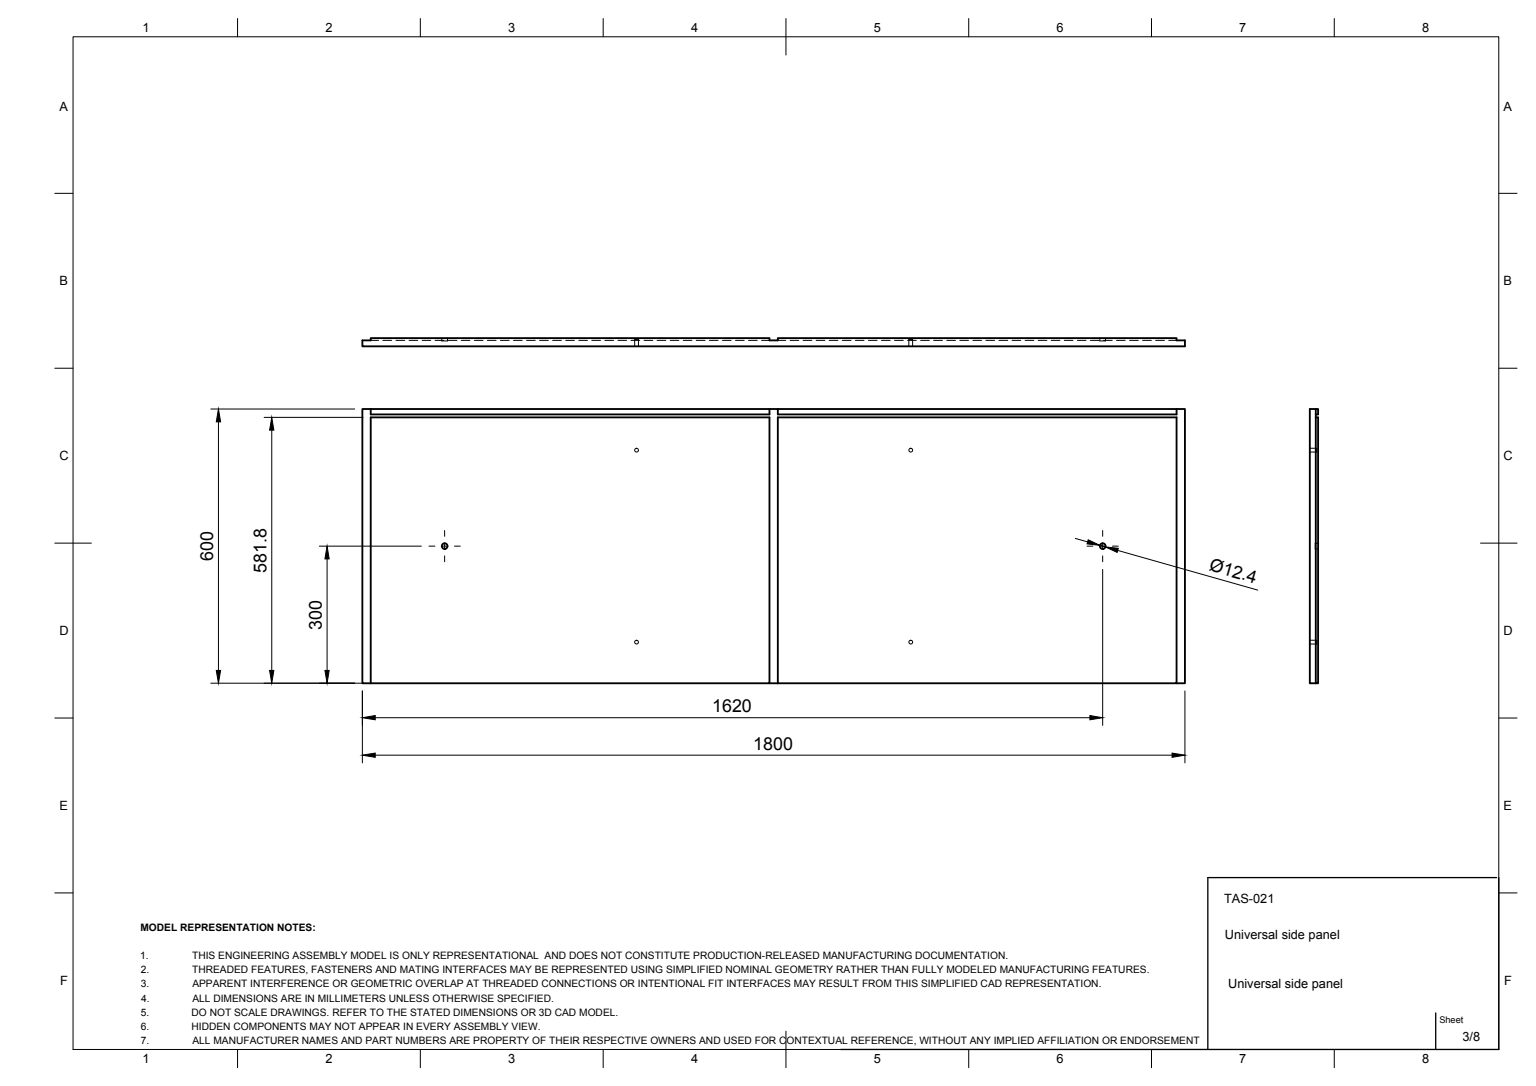
ISO-10303-21;
HEADER;
/* Generated by software containing ST-Developer
 * from STEP Tools, Inc. (www.steptools.com) 
 */

FILE_DESCRIPTION(
/* description */ (''),
/* implementation_level */ '2;1');

FILE_NAME(
/* name */ 'Universal side panel.step',
/* time_stamp */ '2026-11-15T17:48:08-08:00',
/* author */ (''),
/* organization */ (''),
/* preprocessor_version */ 'ST-DEVELOPER v20.2',
/* originating_system */ 'Autodesk Translation Framework v15.17.0.0',
/* authorisation */ '');

FILE_SCHEMA (('AUTOMOTIVE_DESIGN { 1 0 10303 214 3 1 1 }'));
ENDSEC;

DATA;
#10=MECHANICAL_DESIGN_GEOMETRIC_PRESENTATION_REPRESENTATION('',(#139),#2097);
#127=SHAPE_REPRESENTATION_RELATIONSHIP('SRR','None',#2146,#133);
#133=ADVANCED_BREP_SHAPE_REPRESENTATION('',(#145),#2091);
#139=STYLED_ITEM('',(#2185),#145);
#145=MANIFOLD_SOLID_BREP('Body1',#1193);
#151=FACE_BOUND('',#301,.T.);
#152=FACE_BOUND('',#308,.T.);
#153=FACE_BOUND('',#316,.T.);
#154=FACE_BOUND('',#317,.T.);
#155=FACE_BOUND('',#318,.T.);
#156=FACE_BOUND('',#319,.T.);
#159=PLANE('',#1271);
#160=PLANE('',#1275);
#161=PLANE('',#1279);
#162=PLANE('',#1283);
#163=PLANE('',#1287);
#164=PLANE('',#1291);
#165=PLANE('',#1292);
#166=PLANE('',#1293);
#167=PLANE('',#1294);
#168=PLANE('',#1295);
#169=PLANE('',#1296);
#170=PLANE('',#1297);
#171=PLANE('',#1298);
#172=PLANE('',#1299);
#173=PLANE('',#1300);
#174=PLANE('',#1301);
#175=PLANE('',#1302);
#176=PLANE('',#1303);
#177=PLANE('',#1304);
#178=PLANE('',#1305);
#179=PLANE('',#1306);
#180=PLANE('',#1307);
#181=PLANE('',#1308);
#182=PLANE('',#1309);
#183=PLANE('',#1310);
#184=PLANE('',#1311);
#185=PLANE('',#1312);
#186=PLANE('',#1313);
#215=FACE_OUTER_BOUND('',#281,.T.);
#216=FACE_OUTER_BOUND('',#282,.T.);
#217=FACE_OUTER_BOUND('',#283,.T.);
#218=FACE_OUTER_BOUND('',#284,.T.);
#219=FACE_OUTER_BOUND('',#285,.T.);
#220=FACE_OUTER_BOUND('',#286,.T.);
#221=FACE_OUTER_BOUND('',#287,.T.);
#222=FACE_OUTER_BOUND('',#288,.T.);
#223=FACE_OUTER_BOUND('',#289,.T.);
#224=FACE_OUTER_BOUND('',#290,.T.);
#225=FACE_OUTER_BOUND('',#291,.T.);
#226=FACE_OUTER_BOUND('',#292,.T.);
#227=FACE_OUTER_BOUND('',#293,.T.);
#228=FACE_OUTER_BOUND('',#294,.T.);
#229=FACE_OUTER_BOUND('',#295,.T.);
#230=FACE_OUTER_BOUND('',#296,.T.);
#231=FACE_OUTER_BOUND('',#297,.T.);
#232=FACE_OUTER_BOUND('',#298,.T.);
#233=FACE_OUTER_BOUND('',#299,.T.);
#234=FACE_OUTER_BOUND('',#300,.T.);
#235=FACE_OUTER_BOUND('',#302,.T.);
#236=FACE_OUTER_BOUND('',#303,.T.);
#237=FACE_OUTER_BOUND('',#304,.T.);
#238=FACE_OUTER_BOUND('',#305,.T.);
#239=FACE_OUTER_BOUND('',#306,.T.);
#240=FACE_OUTER_BOUND('',#307,.T.);
#241=FACE_OUTER_BOUND('',#309,.T.);
#242=FACE_OUTER_BOUND('',#310,.T.);
#243=FACE_OUTER_BOUND('',#311,.T.);
#244=FACE_OUTER_BOUND('',#312,.T.);
#245=FACE_OUTER_BOUND('',#313,.T.);
#246=FACE_OUTER_BOUND('',#314,.T.);
#247=FACE_OUTER_BOUND('',#315,.T.);
#248=FACE_OUTER_BOUND('',#320,.T.);
#281=EDGE_LOOP('',(#841,#842,#843,#844));
#282=EDGE_LOOP('',(#845));
#283=EDGE_LOOP('',(#846,#847,#848,#849));
#284=EDGE_LOOP('',(#850));
#285=EDGE_LOOP('',(#851,#852,#853,#854));
#286=EDGE_LOOP('',(#855));
#287=EDGE_LOOP('',(#856,#857,#858,#859));
#288=EDGE_LOOP('',(#860));
#289=EDGE_LOOP('',(#861,#862,#863,#864));
#290=EDGE_LOOP('',(#865));
#291=EDGE_LOOP('',(#866,#867,#868,#869));
#292=EDGE_LOOP('',(#870));
#293=EDGE_LOOP('',(#871,#872,#873,#874));
#294=EDGE_LOOP('',(#875,#876,#877,#878));
#295=EDGE_LOOP('',(#879,#880,#881,#882));
#296=EDGE_LOOP('',(#883,#884,#885,#886));
#297=EDGE_LOOP('',(#887,#888,#889,#890,#891,#892,#893,#894,#895,#896,#897,
#898,#899,#900,#901,#902,#903,#904,#905,#906));
#298=EDGE_LOOP('',(#907,#908,#909,#910));
#299=EDGE_LOOP('',(#911,#912,#913,#914));
#300=EDGE_LOOP('',(#915,#916,#917,#918));
#301=EDGE_LOOP('',(#919));
#302=EDGE_LOOP('',(#920,#921,#922,#923));
#303=EDGE_LOOP('',(#924,#925,#926,#927));
#304=EDGE_LOOP('',(#928,#929,#930,#931));
#305=EDGE_LOOP('',(#932,#933,#934,#935));
#306=EDGE_LOOP('',(#936,#937,#938,#939));
#307=EDGE_LOOP('',(#940,#941,#942,#943));
#308=EDGE_LOOP('',(#944));
#309=EDGE_LOOP('',(#945,#946,#947,#948));
#310=EDGE_LOOP('',(#949,#950,#951,#952));
#311=EDGE_LOOP('',(#953,#954,#955,#956));
#312=EDGE_LOOP('',(#957,#958,#959,#960,#961,#962,#963,#964,#965,#966,#967,
#968));
#313=EDGE_LOOP('',(#969,#970,#971,#972));
#314=EDGE_LOOP('',(#973,#974,#975,#976,#977,#978,#979,#980,#981,#982,#983,
#984));
#315=EDGE_LOOP('',(#985,#986,#987,#988));
#316=EDGE_LOOP('',(#989));
#317=EDGE_LOOP('',(#990));
#318=EDGE_LOOP('',(#991));
#319=EDGE_LOOP('',(#992));
#320=EDGE_LOOP('',(#993,#994,#995,#996));
#355=LINE('',#1756,#473);
#356=LINE('',#1763,#474);
#357=LINE('',#1770,#475);
#358=LINE('',#1777,#476);
#359=LINE('',#1784,#477);
#360=LINE('',#1791,#478);
#361=LINE('',#1797,#479);
#362=LINE('',#1799,#480);
#363=LINE('',#1801,#481);
#364=LINE('',#1802,#482);
#365=LINE('',#1806,#483);
#366=LINE('',#1808,#484);
#367=LINE('',#1810,#485);
#368=LINE('',#1811,#486);
#369=LINE('',#1815,#487);
#370=LINE('',#1817,#488);
#371=LINE('',#1819,#489);
#372=LINE('',#1820,#490);
#373=LINE('',#1824,#491);
#374=LINE('',#1826,#492);
#375=LINE('',#1828,#493);
#376=LINE('',#1829,#494);
#377=LINE('',#1832,#495);
#378=LINE('',#1834,#496);
#379=LINE('',#1836,#497);
#380=LINE('',#1838,#498);
#381=LINE('',#1839,#499);
#382=LINE('',#1841,#500);
#383=LINE('',#1843,#501);
#384=LINE('',#1844,#502);
#385=LINE('',#1846,#503);
#386=LINE('',#1848,#504);
#387=LINE('',#1850,#505);
#388=LINE('',#1852,#506);
#389=LINE('',#1853,#507);
#390=LINE('',#1855,#508);
#391=LINE('',#1857,#509);
#392=LINE('',#1858,#510);
#393=LINE('',#1861,#511);
#394=LINE('',#1862,#512);
#395=LINE('',#1865,#513);
#396=LINE('',#1866,#514);
#397=LINE('',#1869,#515);
#398=LINE('',#1870,#516);
#399=LINE('',#1873,#517);
#400=LINE('',#1874,#518);
#401=LINE('',#1876,#519);
#402=LINE('',#1878,#520);
#403=LINE('',#1881,#521);
#404=LINE('',#1882,#522);
#405=LINE('',#1885,#523);
#406=LINE('',#1886,#524);
#407=LINE('',#1889,#525);
#408=LINE('',#1890,#526);
#409=LINE('',#1893,#527);
#410=LINE('',#1894,#528);
#411=LINE('',#1896,#529);
#412=LINE('',#1898,#530);
#413=LINE('',#1901,#531);
#414=LINE('',#1903,#532);
#415=LINE('',#1904,#533);
#416=LINE('',#1907,#534);
#417=LINE('',#1908,#535);
#418=LINE('',#1911,#536);
#419=LINE('',#1912,#537);
#420=LINE('',#1914,#538);
#473=VECTOR('',#1396,0.409999999999997);
#474=VECTOR('',#1405,0.409999999999997);
#475=VECTOR('',#1414,0.409999999999997);
#476=VECTOR('',#1423,0.409999999999997);
#477=VECTOR('',#1432,0.620000000000001);
#478=VECTOR('',#1441,0.620000000000005);
#479=VECTOR('',#1448,1.);
#480=VECTOR('',#1449,1.);
#481=VECTOR('',#1450,1.);
#482=VECTOR('',#1451,1.);
#483=VECTOR('',#1454,1.);
#484=VECTOR('',#1455,1.);
#485=VECTOR('',#1456,1.);
#486=VECTOR('',#1457,1.);
#487=VECTOR('',#1460,1.);
#488=VECTOR('',#1461,1.);
#489=VECTOR('',#1462,1.);
#490=VECTOR('',#1463,1.);
#491=VECTOR('',#1466,1.);
#492=VECTOR('',#1467,1.);
#493=VECTOR('',#1468,1.);
#494=VECTOR('',#1469,1.);
#495=VECTOR('',#1472,1.);
#496=VECTOR('',#1473,1.);
#497=VECTOR('',#1474,1.);
#498=VECTOR('',#1475,1.);
#499=VECTOR('',#1476,1.);
#500=VECTOR('',#1477,1.);
#501=VECTOR('',#1478,1.);
#502=VECTOR('',#1479,1.);
#503=VECTOR('',#1480,1.);
#504=VECTOR('',#1481,1.);
#505=VECTOR('',#1482,1.);
#506=VECTOR('',#1483,1.);
#507=VECTOR('',#1484,1.);
#508=VECTOR('',#1485,1.);
#509=VECTOR('',#1486,1.);
#510=VECTOR('',#1487,1.);
#511=VECTOR('',#1490,1.);
#512=VECTOR('',#1491,1.);
#513=VECTOR('',#1494,1.);
#514=VECTOR('',#1495,1.);
#515=VECTOR('',#1498,1.);
#516=VECTOR('',#1499,1.);
#517=VECTOR('',#1502,1.);
#518=VECTOR('',#1503,1.);
#519=VECTOR('',#1506,1.);
#520=VECTOR('',#1509,1.);
#521=VECTOR('',#1512,1.);
#522=VECTOR('',#1513,1.);
#523=VECTOR('',#1516,1.);
#524=VECTOR('',#1517,1.);
#525=VECTOR('',#1520,1.);
#526=VECTOR('',#1521,1.);
#527=VECTOR('',#1524,1.);
#528=VECTOR('',#1525,1.);
#529=VECTOR('',#1528,1.);
#530=VECTOR('',#1531,1.);
#531=VECTOR('',#1534,1.);
#532=VECTOR('',#1535,1.);
#533=VECTOR('',#1536,1.);
#534=VECTOR('',#1539,1.);
#535=VECTOR('',#1540,1.);
#536=VECTOR('',#1543,1.);
#537=VECTOR('',#1544,1.);
#538=VECTOR('',#1547,1.);
#591=CIRCLE('',#1269,0.409999999999997);
#592=CIRCLE('',#1270,0.409999999999997);
#593=CIRCLE('',#1273,0.409999999999997);
#594=CIRCLE('',#1274,0.409999999999997);
#595=CIRCLE('',#1277,0.409999999999997);
#596=CIRCLE('',#1278,0.409999999999997);
#597=CIRCLE('',#1281,0.409999999999997);
#598=CIRCLE('',#1282,0.409999999999997);
#599=CIRCLE('',#1285,0.620000000000001);
#600=CIRCLE('',#1286,0.620000000000001);
#601=CIRCLE('',#1289,0.620000000000005);
#602=CIRCLE('',#1290,0.620000000000005);
#611=VERTEX_POINT('',#1753);
#612=VERTEX_POINT('',#1755);
#613=VERTEX_POINT('',#1760);
#614=VERTEX_POINT('',#1762);
#615=VERTEX_POINT('',#1767);
#616=VERTEX_POINT('',#1769);
#617=VERTEX_POINT('',#1774);
#618=VERTEX_POINT('',#1776);
#619=VERTEX_POINT('',#1781);
#620=VERTEX_POINT('',#1783);
#621=VERTEX_POINT('',#1788);
#622=VERTEX_POINT('',#1790);
#623=VERTEX_POINT('',#1795);
#624=VERTEX_POINT('',#1796);
#625=VERTEX_POINT('',#1798);
#626=VERTEX_POINT('',#1800);
#627=VERTEX_POINT('',#1804);
#628=VERTEX_POINT('',#1805);
#629=VERTEX_POINT('',#1807);
#630=VERTEX_POINT('',#1809);
#631=VERTEX_POINT('',#1813);
#632=VERTEX_POINT('',#1814);
#633=VERTEX_POINT('',#1816);
#634=VERTEX_POINT('',#1818);
#635=VERTEX_POINT('',#1822);
#636=VERTEX_POINT('',#1823);
#637=VERTEX_POINT('',#1825);
#638=VERTEX_POINT('',#1827);
#639=VERTEX_POINT('',#1831);
#640=VERTEX_POINT('',#1833);
#641=VERTEX_POINT('',#1835);
#642=VERTEX_POINT('',#1837);
#643=VERTEX_POINT('',#1840);
#644=VERTEX_POINT('',#1842);
#645=VERTEX_POINT('',#1845);
#646=VERTEX_POINT('',#1847);
#647=VERTEX_POINT('',#1849);
#648=VERTEX_POINT('',#1851);
#649=VERTEX_POINT('',#1854);
#650=VERTEX_POINT('',#1856);
#651=VERTEX_POINT('',#1860);
#652=VERTEX_POINT('',#1864);
#653=VERTEX_POINT('',#1868);
#654=VERTEX_POINT('',#1872);
#655=VERTEX_POINT('',#1880);
#656=VERTEX_POINT('',#1884);
#657=VERTEX_POINT('',#1888);
#658=VERTEX_POINT('',#1892);
#659=VERTEX_POINT('',#1900);
#660=VERTEX_POINT('',#1902);
#661=VERTEX_POINT('',#1906);
#662=VERTEX_POINT('',#1910);
#703=EDGE_CURVE('',#611,#611,#591,.T.);
#704=EDGE_CURVE('',#611,#612,#355,.T.);
#705=EDGE_CURVE('',#612,#612,#592,.T.);
#706=EDGE_CURVE('',#613,#613,#593,.T.);
#707=EDGE_CURVE('',#613,#614,#356,.T.);
#708=EDGE_CURVE('',#614,#614,#594,.T.);
#709=EDGE_CURVE('',#615,#615,#595,.T.);
#710=EDGE_CURVE('',#615,#616,#357,.T.);
#711=EDGE_CURVE('',#616,#616,#596,.T.);
#712=EDGE_CURVE('',#617,#617,#597,.T.);
#713=EDGE_CURVE('',#617,#618,#358,.T.);
#714=EDGE_CURVE('',#618,#618,#598,.T.);
#715=EDGE_CURVE('',#619,#619,#599,.T.);
#716=EDGE_CURVE('',#619,#620,#359,.T.);
#717=EDGE_CURVE('',#620,#620,#600,.T.);
#718=EDGE_CURVE('',#621,#621,#601,.T.);
#719=EDGE_CURVE('',#621,#622,#360,.T.);
#720=EDGE_CURVE('',#622,#622,#602,.T.);
#721=EDGE_CURVE('',#623,#624,#361,.T.);
#722=EDGE_CURVE('',#625,#623,#362,.T.);
#723=EDGE_CURVE('',#626,#625,#363,.T.);
#724=EDGE_CURVE('',#624,#626,#364,.T.);
#725=EDGE_CURVE('',#627,#628,#365,.T.);
#726=EDGE_CURVE('',#629,#627,#366,.T.);
#727=EDGE_CURVE('',#630,#629,#367,.T.);
#728=EDGE_CURVE('',#628,#630,#368,.T.);
#729=EDGE_CURVE('',#631,#632,#369,.T.);
#730=EDGE_CURVE('',#633,#631,#370,.T.);
#731=EDGE_CURVE('',#634,#633,#371,.T.);
#732=EDGE_CURVE('',#634,#632,#372,.T.);
#733=EDGE_CURVE('',#635,#636,#373,.T.);
#734=EDGE_CURVE('',#637,#635,#374,.T.);
#735=EDGE_CURVE('',#638,#637,#375,.T.);
#736=EDGE_CURVE('',#638,#636,#376,.T.);
#737=EDGE_CURVE('',#639,#627,#377,.T.);
#738=EDGE_CURVE('',#640,#639,#378,.T.);
#739=EDGE_CURVE('',#641,#640,#379,.T.);
#740=EDGE_CURVE('',#642,#641,#380,.T.);
#741=EDGE_CURVE('',#636,#642,#381,.T.);
#742=EDGE_CURVE('',#638,#643,#382,.T.);
#743=EDGE_CURVE('',#644,#643,#383,.T.);
#744=EDGE_CURVE('',#632,#644,#384,.T.);
#745=EDGE_CURVE('',#634,#645,#385,.T.);
#746=EDGE_CURVE('',#646,#645,#386,.T.);
#747=EDGE_CURVE('',#647,#646,#387,.T.);
#748=EDGE_CURVE('',#648,#647,#388,.T.);
#749=EDGE_CURVE('',#648,#625,#389,.T.);
#750=EDGE_CURVE('',#649,#623,#390,.T.);
#751=EDGE_CURVE('',#650,#649,#391,.T.);
#752=EDGE_CURVE('',#650,#629,#392,.T.);
#753=EDGE_CURVE('',#651,#642,#393,.T.);
#754=EDGE_CURVE('',#635,#651,#394,.T.);
#755=EDGE_CURVE('',#652,#628,#395,.T.);
#756=EDGE_CURVE('',#639,#652,#396,.T.);
#757=EDGE_CURVE('',#653,#651,#397,.T.);
#758=EDGE_CURVE('',#653,#637,#398,.T.);
#759=EDGE_CURVE('',#630,#654,#399,.T.);
#760=EDGE_CURVE('',#654,#652,#400,.T.);
#761=EDGE_CURVE('',#643,#653,#401,.T.);
#762=EDGE_CURVE('',#654,#650,#402,.T.);
#763=EDGE_CURVE('',#655,#644,#403,.T.);
#764=EDGE_CURVE('',#631,#655,#404,.T.);
#765=EDGE_CURVE('',#656,#624,#405,.T.);
#766=EDGE_CURVE('',#649,#656,#406,.T.);
#767=EDGE_CURVE('',#657,#655,#407,.T.);
#768=EDGE_CURVE('',#657,#633,#408,.T.);
#769=EDGE_CURVE('',#626,#658,#409,.T.);
#770=EDGE_CURVE('',#658,#656,#410,.T.);
#771=EDGE_CURVE('',#645,#657,#411,.T.);
#772=EDGE_CURVE('',#658,#648,#412,.T.);
#773=EDGE_CURVE('',#647,#659,#413,.T.);
#774=EDGE_CURVE('',#659,#660,#414,.T.);
#775=EDGE_CURVE('',#640,#660,#415,.T.);
#776=EDGE_CURVE('',#661,#646,#416,.T.);
#777=EDGE_CURVE('',#659,#661,#417,.T.);
#778=EDGE_CURVE('',#662,#641,#418,.T.);
#779=EDGE_CURVE('',#661,#662,#419,.T.);
#780=EDGE_CURVE('',#660,#662,#420,.T.);
#841=ORIENTED_EDGE('',*,*,#703,.F.);
#842=ORIENTED_EDGE('',*,*,#704,.T.);
#843=ORIENTED_EDGE('',*,*,#705,.T.);
#844=ORIENTED_EDGE('',*,*,#704,.F.);
#845=ORIENTED_EDGE('',*,*,#705,.F.);
#846=ORIENTED_EDGE('',*,*,#706,.F.);
#847=ORIENTED_EDGE('',*,*,#707,.T.);
#848=ORIENTED_EDGE('',*,*,#708,.T.);
#849=ORIENTED_EDGE('',*,*,#707,.F.);
#850=ORIENTED_EDGE('',*,*,#708,.F.);
#851=ORIENTED_EDGE('',*,*,#709,.F.);
#852=ORIENTED_EDGE('',*,*,#710,.T.);
#853=ORIENTED_EDGE('',*,*,#711,.T.);
#854=ORIENTED_EDGE('',*,*,#710,.F.);
#855=ORIENTED_EDGE('',*,*,#711,.F.);
#856=ORIENTED_EDGE('',*,*,#712,.F.);
#857=ORIENTED_EDGE('',*,*,#713,.T.);
#858=ORIENTED_EDGE('',*,*,#714,.T.);
#859=ORIENTED_EDGE('',*,*,#713,.F.);
#860=ORIENTED_EDGE('',*,*,#714,.F.);
#861=ORIENTED_EDGE('',*,*,#715,.F.);
#862=ORIENTED_EDGE('',*,*,#716,.T.);
#863=ORIENTED_EDGE('',*,*,#717,.T.);
#864=ORIENTED_EDGE('',*,*,#716,.F.);
#865=ORIENTED_EDGE('',*,*,#717,.F.);
#866=ORIENTED_EDGE('',*,*,#718,.F.);
#867=ORIENTED_EDGE('',*,*,#719,.T.);
#868=ORIENTED_EDGE('',*,*,#720,.T.);
#869=ORIENTED_EDGE('',*,*,#719,.F.);
#870=ORIENTED_EDGE('',*,*,#720,.F.);
#871=ORIENTED_EDGE('',*,*,#721,.F.);
#872=ORIENTED_EDGE('',*,*,#722,.F.);
#873=ORIENTED_EDGE('',*,*,#723,.F.);
#874=ORIENTED_EDGE('',*,*,#724,.F.);
#875=ORIENTED_EDGE('',*,*,#725,.F.);
#876=ORIENTED_EDGE('',*,*,#726,.F.);
#877=ORIENTED_EDGE('',*,*,#727,.F.);
#878=ORIENTED_EDGE('',*,*,#728,.F.);
#879=ORIENTED_EDGE('',*,*,#729,.F.);
#880=ORIENTED_EDGE('',*,*,#730,.F.);
#881=ORIENTED_EDGE('',*,*,#731,.F.);
#882=ORIENTED_EDGE('',*,*,#732,.T.);
#883=ORIENTED_EDGE('',*,*,#733,.F.);
#884=ORIENTED_EDGE('',*,*,#734,.F.);
#885=ORIENTED_EDGE('',*,*,#735,.F.);
#886=ORIENTED_EDGE('',*,*,#736,.T.);
#887=ORIENTED_EDGE('',*,*,#737,.F.);
#888=ORIENTED_EDGE('',*,*,#738,.F.);
#889=ORIENTED_EDGE('',*,*,#739,.F.);
#890=ORIENTED_EDGE('',*,*,#740,.F.);
#891=ORIENTED_EDGE('',*,*,#741,.F.);
#892=ORIENTED_EDGE('',*,*,#736,.F.);
#893=ORIENTED_EDGE('',*,*,#742,.T.);
#894=ORIENTED_EDGE('',*,*,#743,.F.);
#895=ORIENTED_EDGE('',*,*,#744,.F.);
#896=ORIENTED_EDGE('',*,*,#732,.F.);
#897=ORIENTED_EDGE('',*,*,#745,.T.);
#898=ORIENTED_EDGE('',*,*,#746,.F.);
#899=ORIENTED_EDGE('',*,*,#747,.F.);
#900=ORIENTED_EDGE('',*,*,#748,.F.);
#901=ORIENTED_EDGE('',*,*,#749,.T.);
#902=ORIENTED_EDGE('',*,*,#722,.T.);
#903=ORIENTED_EDGE('',*,*,#750,.F.);
#904=ORIENTED_EDGE('',*,*,#751,.F.);
#905=ORIENTED_EDGE('',*,*,#752,.T.);
#906=ORIENTED_EDGE('',*,*,#726,.T.);
#907=ORIENTED_EDGE('',*,*,#733,.T.);
#908=ORIENTED_EDGE('',*,*,#741,.T.);
#909=ORIENTED_EDGE('',*,*,#753,.F.);
#910=ORIENTED_EDGE('',*,*,#754,.F.);
#911=ORIENTED_EDGE('',*,*,#725,.T.);
#912=ORIENTED_EDGE('',*,*,#755,.F.);
#913=ORIENTED_EDGE('',*,*,#756,.F.);
#914=ORIENTED_EDGE('',*,*,#737,.T.);
#915=ORIENTED_EDGE('',*,*,#734,.T.);
#916=ORIENTED_EDGE('',*,*,#754,.T.);
#917=ORIENTED_EDGE('',*,*,#757,.F.);
#918=ORIENTED_EDGE('',*,*,#758,.T.);
#919=ORIENTED_EDGE('',*,*,#718,.T.);
#920=ORIENTED_EDGE('',*,*,#728,.T.);
#921=ORIENTED_EDGE('',*,*,#759,.T.);
#922=ORIENTED_EDGE('',*,*,#760,.T.);
#923=ORIENTED_EDGE('',*,*,#755,.T.);
#924=ORIENTED_EDGE('',*,*,#735,.T.);
#925=ORIENTED_EDGE('',*,*,#758,.F.);
#926=ORIENTED_EDGE('',*,*,#761,.F.);
#927=ORIENTED_EDGE('',*,*,#742,.F.);
#928=ORIENTED_EDGE('',*,*,#727,.T.);
#929=ORIENTED_EDGE('',*,*,#752,.F.);
#930=ORIENTED_EDGE('',*,*,#762,.F.);
#931=ORIENTED_EDGE('',*,*,#759,.F.);
#932=ORIENTED_EDGE('',*,*,#729,.T.);
#933=ORIENTED_EDGE('',*,*,#744,.T.);
#934=ORIENTED_EDGE('',*,*,#763,.F.);
#935=ORIENTED_EDGE('',*,*,#764,.F.);
#936=ORIENTED_EDGE('',*,*,#721,.T.);
#937=ORIENTED_EDGE('',*,*,#765,.F.);
#938=ORIENTED_EDGE('',*,*,#766,.F.);
#939=ORIENTED_EDGE('',*,*,#750,.T.);
#940=ORIENTED_EDGE('',*,*,#730,.T.);
#941=ORIENTED_EDGE('',*,*,#764,.T.);
#942=ORIENTED_EDGE('',*,*,#767,.F.);
#943=ORIENTED_EDGE('',*,*,#768,.T.);
#944=ORIENTED_EDGE('',*,*,#715,.T.);
#945=ORIENTED_EDGE('',*,*,#724,.T.);
#946=ORIENTED_EDGE('',*,*,#769,.T.);
#947=ORIENTED_EDGE('',*,*,#770,.T.);
#948=ORIENTED_EDGE('',*,*,#765,.T.);
#949=ORIENTED_EDGE('',*,*,#731,.T.);
#950=ORIENTED_EDGE('',*,*,#768,.F.);
#951=ORIENTED_EDGE('',*,*,#771,.F.);
#952=ORIENTED_EDGE('',*,*,#745,.F.);
#953=ORIENTED_EDGE('',*,*,#723,.T.);
#954=ORIENTED_EDGE('',*,*,#749,.F.);
#955=ORIENTED_EDGE('',*,*,#772,.F.);
#956=ORIENTED_EDGE('',*,*,#769,.F.);
#957=ORIENTED_EDGE('',*,*,#762,.T.);
#958=ORIENTED_EDGE('',*,*,#751,.T.);
#959=ORIENTED_EDGE('',*,*,#766,.T.);
#960=ORIENTED_EDGE('',*,*,#770,.F.);
#961=ORIENTED_EDGE('',*,*,#772,.T.);
#962=ORIENTED_EDGE('',*,*,#748,.T.);
#963=ORIENTED_EDGE('',*,*,#773,.T.);
#964=ORIENTED_EDGE('',*,*,#774,.T.);
#965=ORIENTED_EDGE('',*,*,#775,.F.);
#966=ORIENTED_EDGE('',*,*,#738,.T.);
#967=ORIENTED_EDGE('',*,*,#756,.T.);
#968=ORIENTED_EDGE('',*,*,#760,.F.);
#969=ORIENTED_EDGE('',*,*,#747,.T.);
#970=ORIENTED_EDGE('',*,*,#776,.F.);
#971=ORIENTED_EDGE('',*,*,#777,.F.);
#972=ORIENTED_EDGE('',*,*,#773,.F.);
#973=ORIENTED_EDGE('',*,*,#761,.T.);
#974=ORIENTED_EDGE('',*,*,#757,.T.);
#975=ORIENTED_EDGE('',*,*,#753,.T.);
#976=ORIENTED_EDGE('',*,*,#740,.T.);
#977=ORIENTED_EDGE('',*,*,#778,.F.);
#978=ORIENTED_EDGE('',*,*,#779,.F.);
#979=ORIENTED_EDGE('',*,*,#776,.T.);
#980=ORIENTED_EDGE('',*,*,#746,.T.);
#981=ORIENTED_EDGE('',*,*,#771,.T.);
#982=ORIENTED_EDGE('',*,*,#767,.T.);
#983=ORIENTED_EDGE('',*,*,#763,.T.);
#984=ORIENTED_EDGE('',*,*,#743,.T.);
#985=ORIENTED_EDGE('',*,*,#777,.T.);
#986=ORIENTED_EDGE('',*,*,#779,.T.);
#987=ORIENTED_EDGE('',*,*,#780,.F.);
#988=ORIENTED_EDGE('',*,*,#774,.F.);
#989=ORIENTED_EDGE('',*,*,#703,.T.);
#990=ORIENTED_EDGE('',*,*,#706,.T.);
#991=ORIENTED_EDGE('',*,*,#709,.T.);
#992=ORIENTED_EDGE('',*,*,#712,.T.);
#993=ORIENTED_EDGE('',*,*,#739,.T.);
#994=ORIENTED_EDGE('',*,*,#775,.T.);
#995=ORIENTED_EDGE('',*,*,#780,.T.);
#996=ORIENTED_EDGE('',*,*,#778,.T.);
#1117=CYLINDRICAL_SURFACE('',#1268,0.409999999999997);
#1118=CYLINDRICAL_SURFACE('',#1272,0.409999999999997);
#1119=CYLINDRICAL_SURFACE('',#1276,0.409999999999997);
#1120=CYLINDRICAL_SURFACE('',#1280,0.409999999999997);
#1121=CYLINDRICAL_SURFACE('',#1284,0.620000000000001);
#1122=CYLINDRICAL_SURFACE('',#1288,0.620000000000005);
#1127=ADVANCED_FACE('',(#215),#1117,.F.);
#1128=ADVANCED_FACE('',(#216),#159,.F.);
#1129=ADVANCED_FACE('',(#217),#1118,.F.);
#1130=ADVANCED_FACE('',(#218),#160,.F.);
#1131=ADVANCED_FACE('',(#219),#1119,.F.);
#1132=ADVANCED_FACE('',(#220),#161,.F.);
#1133=ADVANCED_FACE('',(#221),#1120,.F.);
#1134=ADVANCED_FACE('',(#222),#162,.F.);
#1135=ADVANCED_FACE('',(#223),#1121,.F.);
#1136=ADVANCED_FACE('',(#224),#163,.T.);
#1137=ADVANCED_FACE('',(#225),#1122,.F.);
#1138=ADVANCED_FACE('',(#226),#164,.T.);
#1139=ADVANCED_FACE('',(#227),#165,.F.);
#1140=ADVANCED_FACE('',(#228),#166,.F.);
#1141=ADVANCED_FACE('',(#229),#167,.F.);
#1142=ADVANCED_FACE('',(#230),#168,.F.);
#1143=ADVANCED_FACE('',(#231),#169,.F.);
#1144=ADVANCED_FACE('',(#232),#170,.T.);
#1145=ADVANCED_FACE('',(#233),#171,.T.);
#1146=ADVANCED_FACE('',(#234,#151),#172,.T.);
#1147=ADVANCED_FACE('',(#235),#173,.T.);
#1148=ADVANCED_FACE('',(#236),#174,.F.);
#1149=ADVANCED_FACE('',(#237),#175,.F.);
#1150=ADVANCED_FACE('',(#238),#176,.T.);
#1151=ADVANCED_FACE('',(#239),#177,.T.);
#1152=ADVANCED_FACE('',(#240,#152),#178,.T.);
#1153=ADVANCED_FACE('',(#241),#179,.T.);
#1154=ADVANCED_FACE('',(#242),#180,.F.);
#1155=ADVANCED_FACE('',(#243),#181,.F.);
#1156=ADVANCED_FACE('',(#244),#182,.T.);
#1157=ADVANCED_FACE('',(#245),#183,.F.);
#1158=ADVANCED_FACE('',(#246),#184,.T.);
#1159=ADVANCED_FACE('',(#247,#153,#154,#155,#156),#185,.T.);
#1160=ADVANCED_FACE('',(#248),#186,.T.);
#1193=CLOSED_SHELL('',(#1127,#1128,#1129,#1130,#1131,#1132,#1133,#1134,
#1135,#1136,#1137,#1138,#1139,#1140,#1141,#1142,#1143,#1144,#1145,#1146,
#1147,#1148,#1149,#1150,#1151,#1152,#1153,#1154,#1155,#1156,#1157,#1158,
#1159,#1160));
#1267=AXIS2_PLACEMENT_3D('',#1751,#1390,#1391);
#1268=AXIS2_PLACEMENT_3D('',#1752,#1392,#1393);
#1269=AXIS2_PLACEMENT_3D('',#1754,#1394,#1395);
#1270=AXIS2_PLACEMENT_3D('',#1757,#1397,#1398);
#1271=AXIS2_PLACEMENT_3D('',#1758,#1399,#1400);
#1272=AXIS2_PLACEMENT_3D('',#1759,#1401,#1402);
#1273=AXIS2_PLACEMENT_3D('',#1761,#1403,#1404);
#1274=AXIS2_PLACEMENT_3D('',#1764,#1406,#1407);
#1275=AXIS2_PLACEMENT_3D('',#1765,#1408,#1409);
#1276=AXIS2_PLACEMENT_3D('',#1766,#1410,#1411);
#1277=AXIS2_PLACEMENT_3D('',#1768,#1412,#1413);
#1278=AXIS2_PLACEMENT_3D('',#1771,#1415,#1416);
#1279=AXIS2_PLACEMENT_3D('',#1772,#1417,#1418);
#1280=AXIS2_PLACEMENT_3D('',#1773,#1419,#1420);
#1281=AXIS2_PLACEMENT_3D('',#1775,#1421,#1422);
#1282=AXIS2_PLACEMENT_3D('',#1778,#1424,#1425);
#1283=AXIS2_PLACEMENT_3D('',#1779,#1426,#1427);
#1284=AXIS2_PLACEMENT_3D('',#1780,#1428,#1429);
#1285=AXIS2_PLACEMENT_3D('',#1782,#1430,#1431);
#1286=AXIS2_PLACEMENT_3D('',#1785,#1433,#1434);
#1287=AXIS2_PLACEMENT_3D('',#1786,#1435,#1436);
#1288=AXIS2_PLACEMENT_3D('',#1787,#1437,#1438);
#1289=AXIS2_PLACEMENT_3D('',#1789,#1439,#1440);
#1290=AXIS2_PLACEMENT_3D('',#1792,#1442,#1443);
#1291=AXIS2_PLACEMENT_3D('',#1793,#1444,#1445);
#1292=AXIS2_PLACEMENT_3D('',#1794,#1446,#1447);
#1293=AXIS2_PLACEMENT_3D('',#1803,#1452,#1453);
#1294=AXIS2_PLACEMENT_3D('',#1812,#1458,#1459);
#1295=AXIS2_PLACEMENT_3D('',#1821,#1464,#1465);
#1296=AXIS2_PLACEMENT_3D('',#1830,#1470,#1471);
#1297=AXIS2_PLACEMENT_3D('',#1859,#1488,#1489);
#1298=AXIS2_PLACEMENT_3D('',#1863,#1492,#1493);
#1299=AXIS2_PLACEMENT_3D('',#1867,#1496,#1497);
#1300=AXIS2_PLACEMENT_3D('',#1871,#1500,#1501);
#1301=AXIS2_PLACEMENT_3D('',#1875,#1504,#1505);
#1302=AXIS2_PLACEMENT_3D('',#1877,#1507,#1508);
#1303=AXIS2_PLACEMENT_3D('',#1879,#1510,#1511);
#1304=AXIS2_PLACEMENT_3D('',#1883,#1514,#1515);
#1305=AXIS2_PLACEMENT_3D('',#1887,#1518,#1519);
#1306=AXIS2_PLACEMENT_3D('',#1891,#1522,#1523);
#1307=AXIS2_PLACEMENT_3D('',#1895,#1526,#1527);
#1308=AXIS2_PLACEMENT_3D('',#1897,#1529,#1530);
#1309=AXIS2_PLACEMENT_3D('',#1899,#1532,#1533);
#1310=AXIS2_PLACEMENT_3D('',#1905,#1537,#1538);
#1311=AXIS2_PLACEMENT_3D('',#1909,#1541,#1542);
#1312=AXIS2_PLACEMENT_3D('',#1913,#1545,#1546);
#1313=AXIS2_PLACEMENT_3D('',#1915,#1548,#1549);
#1390=DIRECTION('axis',(0.,0.,1.));
#1391=DIRECTION('refdir',(1.,0.,0.));
#1392=DIRECTION('center_axis',(1.,0.,0.));
#1393=DIRECTION('ref_axis',(0.,0.,-1.));
#1394=DIRECTION('center_axis',(1.,0.,0.));
#1395=DIRECTION('ref_axis',(0.,0.,-1.));
#1396=DIRECTION('',(1.,0.,0.));
#1397=DIRECTION('center_axis',(1.,0.,0.));
#1398=DIRECTION('ref_axis',(0.,0.,-1.));
#1399=DIRECTION('center_axis',(1.,0.,0.));
#1400=DIRECTION('ref_axis',(0.,0.,-1.));
#1401=DIRECTION('center_axis',(1.,0.,0.));
#1402=DIRECTION('ref_axis',(0.,0.,-1.));
#1403=DIRECTION('center_axis',(1.,0.,0.));
#1404=DIRECTION('ref_axis',(0.,0.,-1.));
#1405=DIRECTION('',(1.,0.,0.));
#1406=DIRECTION('center_axis',(1.,0.,0.));
#1407=DIRECTION('ref_axis',(0.,0.,-1.));
#1408=DIRECTION('center_axis',(1.,0.,0.));
#1409=DIRECTION('ref_axis',(0.,0.,-1.));
#1410=DIRECTION('center_axis',(1.,0.,0.));
#1411=DIRECTION('ref_axis',(0.,0.,-1.));
#1412=DIRECTION('center_axis',(1.,0.,0.));
#1413=DIRECTION('ref_axis',(0.,0.,-1.));
#1414=DIRECTION('',(1.,0.,0.));
#1415=DIRECTION('center_axis',(1.,0.,0.));
#1416=DIRECTION('ref_axis',(0.,0.,-1.));
#1417=DIRECTION('center_axis',(1.,0.,0.));
#1418=DIRECTION('ref_axis',(0.,0.,-1.));
#1419=DIRECTION('center_axis',(1.,0.,0.));
#1420=DIRECTION('ref_axis',(0.,0.,-1.));
#1421=DIRECTION('center_axis',(1.,0.,0.));
#1422=DIRECTION('ref_axis',(0.,0.,-1.));
#1423=DIRECTION('',(1.,0.,0.));
#1424=DIRECTION('center_axis',(1.,0.,0.));
#1425=DIRECTION('ref_axis',(0.,0.,-1.));
#1426=DIRECTION('center_axis',(1.,0.,0.));
#1427=DIRECTION('ref_axis',(0.,0.,-1.));
#1428=DIRECTION('center_axis',(-1.,0.,0.));
#1429=DIRECTION('ref_axis',(0.,0.,-1.));
#1430=DIRECTION('center_axis',(-1.,0.,0.));
#1431=DIRECTION('ref_axis',(0.,0.,-1.));
#1432=DIRECTION('',(-1.,0.,0.));
#1433=DIRECTION('center_axis',(-1.,0.,0.));
#1434=DIRECTION('ref_axis',(0.,0.,-1.));
#1435=DIRECTION('center_axis',(1.,0.,0.));
#1436=DIRECTION('ref_axis',(0.,0.,-1.));
#1437=DIRECTION('center_axis',(-1.,0.,0.));
#1438=DIRECTION('ref_axis',(0.,0.,-1.));
#1439=DIRECTION('center_axis',(-1.,0.,0.));
#1440=DIRECTION('ref_axis',(0.,0.,-1.));
#1441=DIRECTION('',(-1.,0.,0.));
#1442=DIRECTION('center_axis',(-1.,0.,0.));
#1443=DIRECTION('ref_axis',(0.,0.,-1.));
#1444=DIRECTION('center_axis',(1.,0.,0.));
#1445=DIRECTION('ref_axis',(0.,0.,-1.));
#1446=DIRECTION('center_axis',(0.,1.,0.));
#1447=DIRECTION('ref_axis',(-1.,0.,0.));
#1448=DIRECTION('',(1.,0.,0.));
#1449=DIRECTION('',(0.,0.,1.));
#1450=DIRECTION('',(-1.,0.,0.));
#1451=DIRECTION('',(0.,0.,-1.));
#1452=DIRECTION('center_axis',(0.,1.,0.));
#1453=DIRECTION('ref_axis',(-1.,0.,0.));
#1454=DIRECTION('',(1.,0.,0.));
#1455=DIRECTION('',(0.,0.,1.));
#1456=DIRECTION('',(-1.,0.,0.));
#1457=DIRECTION('',(0.,0.,-1.));
#1458=DIRECTION('center_axis',(0.,-1.,0.));
#1459=DIRECTION('ref_axis',(1.,0.,0.));
#1460=DIRECTION('',(-1.,0.,0.));
#1461=DIRECTION('',(0.,0.,1.));
#1462=DIRECTION('',(1.,0.,0.));
#1463=DIRECTION('',(0.,0.,1.));
#1464=DIRECTION('center_axis',(0.,-1.,0.));
#1465=DIRECTION('ref_axis',(1.,0.,0.));
#1466=DIRECTION('',(-1.,0.,0.));
#1467=DIRECTION('',(0.,0.,1.));
#1468=DIRECTION('',(1.,0.,0.));
#1469=DIRECTION('',(0.,0.,1.));
#1470=DIRECTION('center_axis',(-1.,0.,0.));
#1471=DIRECTION('ref_axis',(0.,-1.,0.));
#1472=DIRECTION('',(0.,-1.,0.));
#1473=DIRECTION('',(0.,0.,-1.));
#1474=DIRECTION('',(0.,1.,0.));
#1475=DIRECTION('',(0.,0.,1.));
#1476=DIRECTION('',(0.,-1.,0.));
#1477=DIRECTION('',(0.,-1.,0.));
#1478=DIRECTION('',(0.,0.,1.));
#1479=DIRECTION('',(0.,-1.,0.));
#1480=DIRECTION('',(0.,-1.,0.));
#1481=DIRECTION('',(0.,0.,1.));
#1482=DIRECTION('',(0.,-1.,0.));
#1483=DIRECTION('',(0.,0.,-1.));
#1484=DIRECTION('',(0.,-1.,0.));
#1485=DIRECTION('',(0.,-1.,0.));
#1486=DIRECTION('',(0.,0.,-1.));
#1487=DIRECTION('',(0.,-1.,0.));
#1488=DIRECTION('center_axis',(0.,0.,1.));
#1489=DIRECTION('ref_axis',(1.,0.,0.));
#1490=DIRECTION('',(-1.,0.,0.));
#1491=DIRECTION('',(0.,-1.,0.));
#1492=DIRECTION('center_axis',(0.,0.,1.));
#1493=DIRECTION('ref_axis',(1.,0.,0.));
#1494=DIRECTION('',(0.,-1.,0.));
#1495=DIRECTION('',(1.,0.,0.));
#1496=DIRECTION('center_axis',(1.,0.,0.));
#1497=DIRECTION('ref_axis',(0.,1.,0.));
#1498=DIRECTION('',(0.,0.,1.));
#1499=DIRECTION('',(0.,1.,0.));
#1500=DIRECTION('center_axis',(1.,0.,0.));
#1501=DIRECTION('ref_axis',(0.,1.,0.));
#1502=DIRECTION('',(0.,1.,0.));
#1503=DIRECTION('',(0.,0.,1.));
#1504=DIRECTION('center_axis',(0.,0.,1.));
#1505=DIRECTION('ref_axis',(1.,0.,0.));
#1506=DIRECTION('',(1.,0.,0.));
#1507=DIRECTION('center_axis',(0.,0.,1.));
#1508=DIRECTION('ref_axis',(1.,0.,0.));
#1509=DIRECTION('',(-1.,0.,0.));
#1510=DIRECTION('center_axis',(0.,0.,1.));
#1511=DIRECTION('ref_axis',(1.,0.,0.));
#1512=DIRECTION('',(-1.,0.,0.));
#1513=DIRECTION('',(0.,-1.,0.));
#1514=DIRECTION('center_axis',(0.,0.,1.));
#1515=DIRECTION('ref_axis',(1.,0.,0.));
#1516=DIRECTION('',(0.,-1.,0.));
#1517=DIRECTION('',(1.,0.,0.));
#1518=DIRECTION('center_axis',(1.,0.,0.));
#1519=DIRECTION('ref_axis',(0.,1.,0.));
#1520=DIRECTION('',(0.,0.,1.));
#1521=DIRECTION('',(0.,1.,0.));
#1522=DIRECTION('center_axis',(1.,0.,0.));
#1523=DIRECTION('ref_axis',(0.,1.,0.));
#1524=DIRECTION('',(0.,1.,0.));
#1525=DIRECTION('',(0.,0.,1.));
#1526=DIRECTION('center_axis',(0.,0.,1.));
#1527=DIRECTION('ref_axis',(1.,0.,0.));
#1528=DIRECTION('',(1.,0.,0.));
#1529=DIRECTION('center_axis',(0.,0.,1.));
#1530=DIRECTION('ref_axis',(1.,0.,0.));
#1531=DIRECTION('',(-1.,0.,0.));
#1532=DIRECTION('center_axis',(0.,1.,0.));
#1533=DIRECTION('ref_axis',(-1.,0.,0.));
#1534=DIRECTION('',(-1.,0.,0.));
#1535=DIRECTION('',(0.,0.,1.));
#1536=DIRECTION('',(-1.,0.,0.));
#1537=DIRECTION('center_axis',(0.,0.,1.));
#1538=DIRECTION('ref_axis',(1.,0.,0.));
#1539=DIRECTION('',(1.,0.,0.));
#1540=DIRECTION('',(0.,-1.,0.));
#1541=DIRECTION('center_axis',(0.,-1.,0.));
#1542=DIRECTION('ref_axis',(1.,0.,0.));
#1543=DIRECTION('',(1.,0.,0.));
#1544=DIRECTION('',(0.,0.,1.));
#1545=DIRECTION('center_axis',(-1.,0.,0.));
#1546=DIRECTION('ref_axis',(0.,-1.,0.));
#1547=DIRECTION('',(0.,-1.,0.));
#1548=DIRECTION('center_axis',(0.,0.,1.));
#1549=DIRECTION('ref_axis',(1.,0.,0.));
#1751=CARTESIAN_POINT('',(0.,0.,0.));
#1752=CARTESIAN_POINT('Origin',(0.,51.,60.));
#1753=CARTESIAN_POINT('',(0.,51.,60.41));
#1754=CARTESIAN_POINT('Origin',(0.,51.,60.));
#1755=CARTESIAN_POINT('',(1.5,51.,60.41));
#1756=CARTESIAN_POINT('',(0.,51.,60.41));
#1757=CARTESIAN_POINT('Origin',(1.5,51.,60.));
#1758=CARTESIAN_POINT('Origin',(1.5,51.,60.));
#1759=CARTESIAN_POINT('Origin',(0.,9.,120.));
#1760=CARTESIAN_POINT('',(0.,9.,120.41));
#1761=CARTESIAN_POINT('Origin',(0.,9.,120.));
#1762=CARTESIAN_POINT('',(1.5,9.,120.41));
#1763=CARTESIAN_POINT('',(0.,9.,120.41));
#1764=CARTESIAN_POINT('Origin',(1.5,9.,120.));
#1765=CARTESIAN_POINT('Origin',(1.5,9.,120.));
#1766=CARTESIAN_POINT('Origin',(0.,9.,60.));
#1767=CARTESIAN_POINT('',(0.,9.,60.41));
#1768=CARTESIAN_POINT('Origin',(0.,9.,60.));
#1769=CARTESIAN_POINT('',(1.5,9.,60.41));
#1770=CARTESIAN_POINT('',(0.,9.,60.41));
#1771=CARTESIAN_POINT('Origin',(1.5,9.,60.));
#1772=CARTESIAN_POINT('Origin',(1.5,9.,60.));
#1773=CARTESIAN_POINT('Origin',(0.,51.,120.));
#1774=CARTESIAN_POINT('',(0.,51.,120.41));
#1775=CARTESIAN_POINT('Origin',(0.,51.,120.));
#1776=CARTESIAN_POINT('',(1.5,51.,120.41));
#1777=CARTESIAN_POINT('',(0.,51.,120.41));
#1778=CARTESIAN_POINT('Origin',(1.5,51.,120.));
#1779=CARTESIAN_POINT('Origin',(1.5,51.,120.));
#1780=CARTESIAN_POINT('Origin',(1.8,30.,18.));
#1781=CARTESIAN_POINT('',(1.8,30.,18.62));
#1782=CARTESIAN_POINT('Origin',(1.8,30.,18.));
#1783=CARTESIAN_POINT('',(1.18,30.,18.62));
#1784=CARTESIAN_POINT('',(1.8,30.,18.62));
#1785=CARTESIAN_POINT('Origin',(1.18,30.,18.));
#1786=CARTESIAN_POINT('Origin',(1.18,30.,18.));
#1787=CARTESIAN_POINT('Origin',(1.8,30.,162.));
#1788=CARTESIAN_POINT('',(1.8,30.,162.62));
#1789=CARTESIAN_POINT('Origin',(1.8,30.,162.));
#1790=CARTESIAN_POINT('',(1.18,30.,162.62));
#1791=CARTESIAN_POINT('',(1.8,30.,162.62));
#1792=CARTESIAN_POINT('Origin',(1.18,30.,162.));
#1793=CARTESIAN_POINT('Origin',(1.18,30.,162.));
#1794=CARTESIAN_POINT('Origin',(1.81,58.82,0.));
#1795=CARTESIAN_POINT('',(1.3,58.82,89.08));
#1796=CARTESIAN_POINT('',(1.8,58.82,89.08));
#1797=CARTESIAN_POINT('',(1.6825,58.82,89.08));
#1798=CARTESIAN_POINT('',(1.3,58.82,1.82));
#1799=CARTESIAN_POINT('',(1.3,58.82,0.));
#1800=CARTESIAN_POINT('',(1.8,58.82,1.82));
#1801=CARTESIAN_POINT('',(1.6825,58.82,1.82));
#1802=CARTESIAN_POINT('',(1.8,58.82,0.));
#1803=CARTESIAN_POINT('Origin',(1.81,58.82,0.));
#1804=CARTESIAN_POINT('',(1.3,58.82,178.18));
#1805=CARTESIAN_POINT('',(1.8,58.82,178.18));
#1806=CARTESIAN_POINT('',(1.6825,58.82,178.18));
#1807=CARTESIAN_POINT('',(1.3,58.82,90.92));
#1808=CARTESIAN_POINT('',(1.3,58.82,0.));
#1809=CARTESIAN_POINT('',(1.8,58.82,90.92));
#1810=CARTESIAN_POINT('',(1.6825,58.82,90.92));
#1811=CARTESIAN_POINT('',(1.8,58.82,0.));
#1812=CARTESIAN_POINT('Origin',(1.3,58.18,0.));
#1813=CARTESIAN_POINT('',(1.8,58.18,89.08));
#1814=CARTESIAN_POINT('',(1.3,58.18,89.08));
#1815=CARTESIAN_POINT('',(1.4275,58.18,89.08));
#1816=CARTESIAN_POINT('',(1.8,58.18,1.82));
#1817=CARTESIAN_POINT('',(1.8,58.18,0.));
#1818=CARTESIAN_POINT('',(1.3,58.18,1.82));
#1819=CARTESIAN_POINT('',(1.4275,58.18,1.82));
#1820=CARTESIAN_POINT('',(1.3,58.18,0.));
#1821=CARTESIAN_POINT('Origin',(1.3,58.18,0.));
#1822=CARTESIAN_POINT('',(1.8,58.18,178.18));
#1823=CARTESIAN_POINT('',(1.3,58.18,178.18));
#1824=CARTESIAN_POINT('',(1.4275,58.18,178.18));
#1825=CARTESIAN_POINT('',(1.8,58.18,90.92));
#1826=CARTESIAN_POINT('',(1.8,58.18,0.));
#1827=CARTESIAN_POINT('',(1.3,58.18,90.92));
#1828=CARTESIAN_POINT('',(1.4275,58.18,90.92));
#1829=CARTESIAN_POINT('',(1.3,58.18,0.));
#1830=CARTESIAN_POINT('Origin',(1.3,60.,178.18));
#1831=CARTESIAN_POINT('',(1.3,60.,178.18));
#1832=CARTESIAN_POINT('',(1.3,60.,178.18));
#1833=CARTESIAN_POINT('',(1.3,60.,180.));
#1834=CARTESIAN_POINT('',(1.3,60.,89.09));
#1835=CARTESIAN_POINT('',(1.3,0.,180.));
#1836=CARTESIAN_POINT('',(1.3,45.,180.));
#1837=CARTESIAN_POINT('',(1.3,0.,178.18));
#1838=CARTESIAN_POINT('',(1.3,0.,89.09));
#1839=CARTESIAN_POINT('',(1.3,60.,178.18));
#1840=CARTESIAN_POINT('',(1.3,0.,90.92));
#1841=CARTESIAN_POINT('',(1.3,60.,90.92));
#1842=CARTESIAN_POINT('',(1.3,0.,89.08));
#1843=CARTESIAN_POINT('',(1.3,0.,44.54));
#1844=CARTESIAN_POINT('',(1.3,60.,89.08));
#1845=CARTESIAN_POINT('',(1.3,0.,1.82));
#1846=CARTESIAN_POINT('',(1.3,60.,1.82));
#1847=CARTESIAN_POINT('',(1.3,0.,0.));
#1848=CARTESIAN_POINT('',(1.3,0.,0.));
#1849=CARTESIAN_POINT('',(1.3,60.,0.));
#1850=CARTESIAN_POINT('',(1.3,45.,0.));
#1851=CARTESIAN_POINT('',(1.3,60.,1.82));
#1852=CARTESIAN_POINT('',(1.3,60.,0.));
#1853=CARTESIAN_POINT('',(1.3,60.,1.82));
#1854=CARTESIAN_POINT('',(1.3,60.,89.08));
#1855=CARTESIAN_POINT('',(1.3,60.,89.08));
#1856=CARTESIAN_POINT('',(1.3,60.,90.92));
#1857=CARTESIAN_POINT('',(1.3,60.,44.54));
#1858=CARTESIAN_POINT('',(1.3,60.,90.92));
#1859=CARTESIAN_POINT('Origin',(1.555,30.,178.18));
#1860=CARTESIAN_POINT('',(1.8,0.,178.18));
#1861=CARTESIAN_POINT('',(0.7775,0.,178.18));
#1862=CARTESIAN_POINT('',(1.8,15.,178.18));
#1863=CARTESIAN_POINT('Origin',(1.555,30.,178.18));
#1864=CARTESIAN_POINT('',(1.8,60.,178.18));
#1865=CARTESIAN_POINT('',(1.8,15.,178.18));
#1866=CARTESIAN_POINT('',(1.6775,60.,178.18));
#1867=CARTESIAN_POINT('Origin',(1.8,0.,0.));
#1868=CARTESIAN_POINT('',(1.8,0.,90.92));
#1869=CARTESIAN_POINT('',(1.8,0.,0.));
#1870=CARTESIAN_POINT('',(1.8,15.,90.92));
#1871=CARTESIAN_POINT('Origin',(1.8,0.,0.));
#1872=CARTESIAN_POINT('',(1.8,60.,90.92));
#1873=CARTESIAN_POINT('',(1.8,15.,90.92));
#1874=CARTESIAN_POINT('',(1.8,60.,0.));
#1875=CARTESIAN_POINT('Origin',(1.555,30.,90.92));
#1876=CARTESIAN_POINT('',(0.7775,0.,90.92));
#1877=CARTESIAN_POINT('Origin',(1.555,30.,90.92));
#1878=CARTESIAN_POINT('',(1.6775,60.,90.92));
#1879=CARTESIAN_POINT('Origin',(1.555,30.,89.08));
#1880=CARTESIAN_POINT('',(1.8,0.,89.08));
#1881=CARTESIAN_POINT('',(0.7775,0.,89.08));
#1882=CARTESIAN_POINT('',(1.8,15.,89.08));
#1883=CARTESIAN_POINT('Origin',(1.555,30.,89.08));
#1884=CARTESIAN_POINT('',(1.8,60.,89.08));
#1885=CARTESIAN_POINT('',(1.8,15.,89.08));
#1886=CARTESIAN_POINT('',(1.6775,60.,89.08));
#1887=CARTESIAN_POINT('Origin',(1.8,0.,0.));
#1888=CARTESIAN_POINT('',(1.8,0.,1.82));
#1889=CARTESIAN_POINT('',(1.8,0.,0.));
#1890=CARTESIAN_POINT('',(1.8,15.,1.82));
#1891=CARTESIAN_POINT('Origin',(1.8,0.,0.));
#1892=CARTESIAN_POINT('',(1.8,60.,1.82));
#1893=CARTESIAN_POINT('',(1.8,15.,1.82));
#1894=CARTESIAN_POINT('',(1.8,60.,0.));
#1895=CARTESIAN_POINT('Origin',(1.555,30.,1.82));
#1896=CARTESIAN_POINT('',(0.7775,0.,1.82));
#1897=CARTESIAN_POINT('Origin',(1.555,30.,1.82));
#1898=CARTESIAN_POINT('',(1.6775,60.,1.82));
#1899=CARTESIAN_POINT('Origin',(1.8,60.,0.));
#1900=CARTESIAN_POINT('',(0.,60.,0.));
#1901=CARTESIAN_POINT('',(1.8,60.,0.));
#1902=CARTESIAN_POINT('',(0.,60.,180.));
#1903=CARTESIAN_POINT('',(0.,60.,0.));
#1904=CARTESIAN_POINT('',(1.8,60.,180.));
#1905=CARTESIAN_POINT('Origin',(0.9,30.,0.));
#1906=CARTESIAN_POINT('',(0.,0.,0.));
#1907=CARTESIAN_POINT('',(0.,0.,0.));
#1908=CARTESIAN_POINT('',(0.,60.,0.));
#1909=CARTESIAN_POINT('Origin',(0.,0.,0.));
#1910=CARTESIAN_POINT('',(0.,0.,180.));
#1911=CARTESIAN_POINT('',(0.,0.,180.));
#1912=CARTESIAN_POINT('',(0.,0.,0.));
#1913=CARTESIAN_POINT('Origin',(0.,60.,0.));
#1914=CARTESIAN_POINT('',(0.,60.,180.));
#1915=CARTESIAN_POINT('Origin',(0.9,30.,180.));
#2083=UNCERTAINTY_MEASURE_WITH_UNIT(LENGTH_MEASURE(0.001),#2098,
'DISTANCE_ACCURACY_VALUE',
'Maximum model space distance between geometric entities at asserted c
onnectivities');
#2089=UNCERTAINTY_MEASURE_WITH_UNIT(LENGTH_MEASURE(0.001),#2098,
'DISTANCE_ACCURACY_VALUE',
'Maximum model space distance between geometric entities at asserted c
onnectivities');
#2091=(
GEOMETRIC_REPRESENTATION_CONTEXT(3)
GLOBAL_UNCERTAINTY_ASSIGNED_CONTEXT((#2083))
GLOBAL_UNIT_ASSIGNED_CONTEXT((#2098,#2100,#2101))
REPRESENTATION_CONTEXT('','3D')
);
#2097=(
GEOMETRIC_REPRESENTATION_CONTEXT(3)
GLOBAL_UNCERTAINTY_ASSIGNED_CONTEXT((#2089))
GLOBAL_UNIT_ASSIGNED_CONTEXT((#2098,#2100,#2101))
REPRESENTATION_CONTEXT('','3D')
);
#2098=(
LENGTH_UNIT()
NAMED_UNIT(*)
SI_UNIT(.CENTI.,.METRE.)
);
#2100=(
NAMED_UNIT(*)
PLANE_ANGLE_UNIT()
SI_UNIT($,.RADIAN.)
);
#2101=(
NAMED_UNIT(*)
SI_UNIT($,.STERADIAN.)
SOLID_ANGLE_UNIT()
);
#2103=SHAPE_DEFINITION_REPRESENTATION(#2110,#2146);
#2110=PRODUCT_DEFINITION_SHAPE('',$,#2154);
#2146=SHAPE_REPRESENTATION('',(#1267),#2091);
#2152=PRODUCT_DEFINITION_CONTEXT('part definition',#2175,'design');
#2154=PRODUCT_DEFINITION('Universal side panel','Universal side panel',
#2161,#2152);
#2161=PRODUCT_DEFINITION_FORMATION('',$,#2178);
#2175=APPLICATION_CONTEXT(
'Core Data for Automotive Mechanical Design Process');
#2176=PRODUCT_CONTEXT('part definition',#2175,'mechanical');
#2178=PRODUCT('Universal side panel','Universal side panel',$,(#2176));
#2185=PRESENTATION_STYLE_ASSIGNMENT((#2192));
#2192=SURFACE_STYLE_USAGE(.BOTH.,#2199);
#2199=SURFACE_SIDE_STYLE('',(#2206));
#2206=SURFACE_STYLE_FILL_AREA(#2213);
#2213=FILL_AREA_STYLE('Universal side panel finish',(#2220));
#2220=FILL_AREA_STYLE_COLOUR('Universal side panel finish',#2227);
#2227=COLOUR_RGB('Universal side panel finish',0.0941176470588235,0.231372549019608,
0.431372549019608);
ENDSEC;
END-ISO-10303-21;
